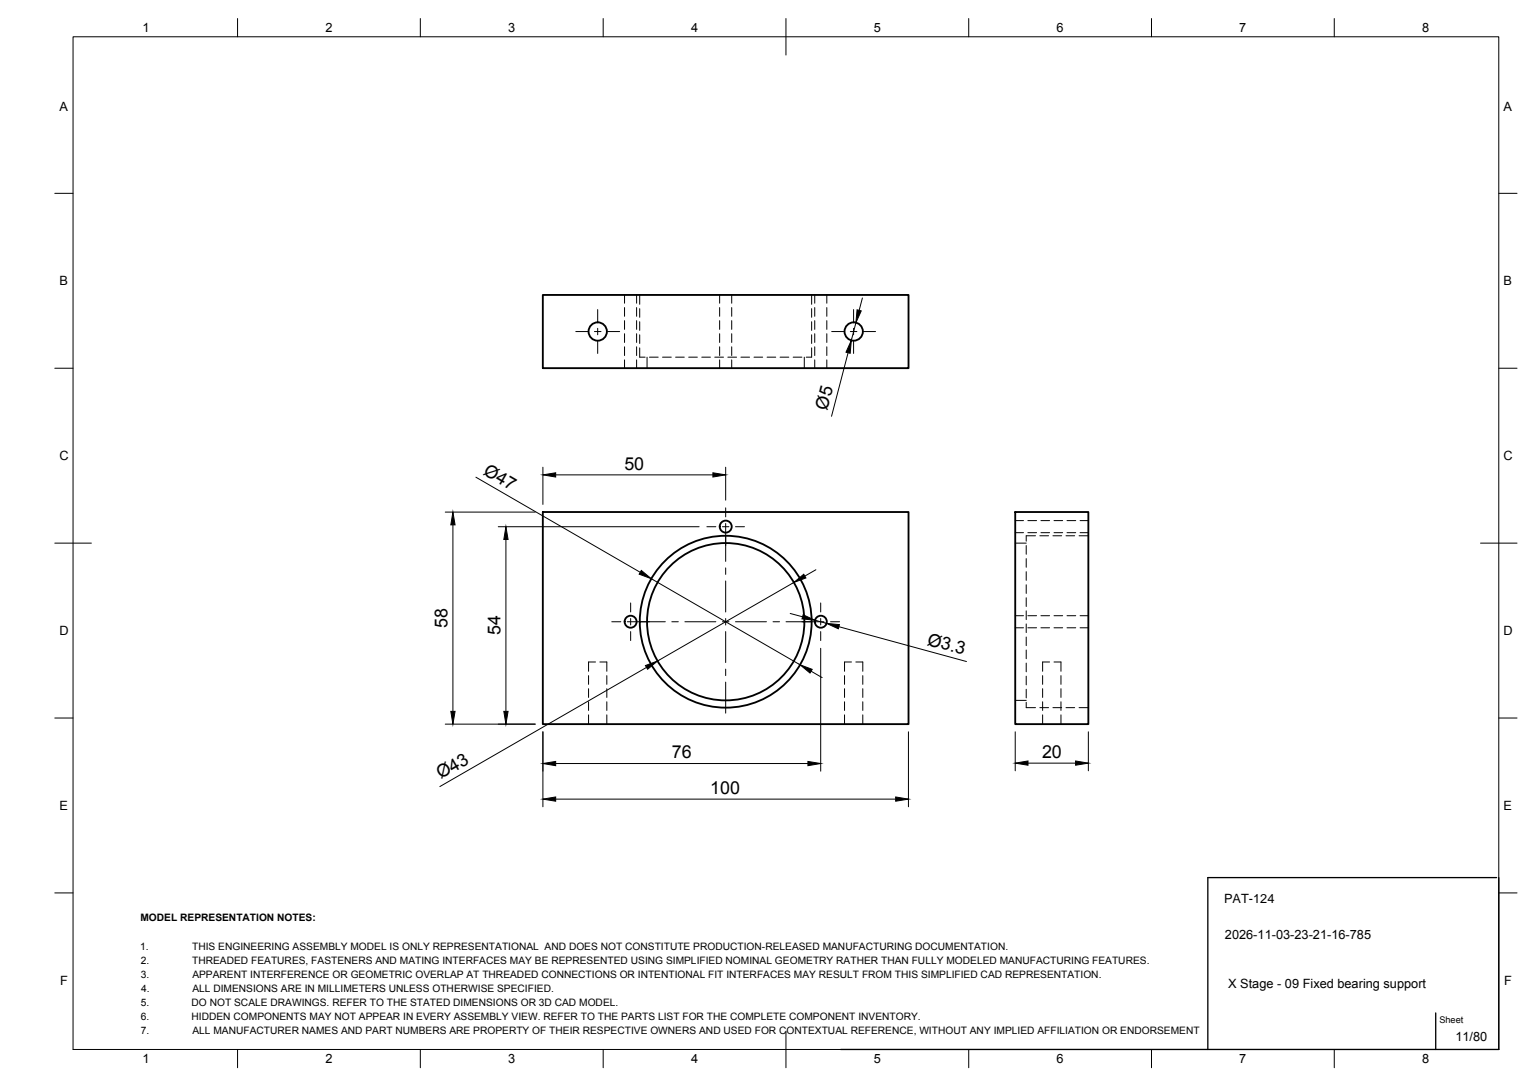
ISO-10303-21;
HEADER;
/* Generated by software containing ST-Developer
 * from STEP Tools, Inc. (www.steptools.com) 
 */

FILE_DESCRIPTION(
/* description */ ('XY cross-slide table'),
/* implementation_level */ '2;1');

FILE_NAME(
/* name */ 'X Stage - 09 Fixed bearing support.step',
/* time_stamp */ '2026-10-28T03:22:46-07:00',
/* author */ (''),
/* organization */ (''),
/* preprocessor_version */ 'ST-DEVELOPER v20.2',
/* originating_system */ 'Autodesk Translation Framework v15.17.0.0',
/* authorisation */ '');

FILE_SCHEMA (('AUTOMOTIVE_DESIGN { 1 0 10303 214 3 1 1 }'));
ENDSEC;

DATA;
#10=MECHANICAL_DESIGN_GEOMETRIC_PRESENTATION_REPRESENTATION('',(#1676),#62984);
#1510=SHAPE_REPRESENTATION_RELATIONSHIP('SRR','None',#63358,#1593);
#1593=ADVANCED_BREP_SHAPE_REPRESENTATION('',(#1789),#62895);
#1676=STYLED_ITEM('',(#63912),#1789);
#1789=MANIFOLD_SOLID_BREP('Body1',#22970);
#1945=FACE_BOUND('',#4323,.T.);
#1946=FACE_BOUND('',#4331,.T.);
#1947=FACE_BOUND('',#4332,.T.);
#1948=FACE_BOUND('',#4333,.T.);
#1949=FACE_BOUND('',#4334,.T.);
#1950=FACE_BOUND('',#4337,.T.);
#1951=FACE_BOUND('',#4338,.T.);
#1952=FACE_BOUND('',#4339,.T.);
#1953=FACE_BOUND('',#4340,.T.);
#1954=FACE_BOUND('',#4343,.T.);
#1955=FACE_BOUND('',#4344,.T.);
#2336=PLANE('',#24173);
#2337=PLANE('',#24180);
#2338=PLANE('',#24184);
#2339=PLANE('',#24185);
#2340=PLANE('',#24186);
#2341=PLANE('',#24187);
#2342=PLANE('',#24188);
#2343=PLANE('',#24189);
#2344=PLANE('',#24190);
#2946=FACE_OUTER_BOUND('',#4318,.T.);
#2947=FACE_OUTER_BOUND('',#4319,.T.);
#2948=FACE_OUTER_BOUND('',#4320,.T.);
#2949=FACE_OUTER_BOUND('',#4321,.T.);
#2950=FACE_OUTER_BOUND('',#4322,.T.);
#2951=FACE_OUTER_BOUND('',#4324,.T.);
#2952=FACE_OUTER_BOUND('',#4325,.T.);
#2953=FACE_OUTER_BOUND('',#4326,.T.);
#2954=FACE_OUTER_BOUND('',#4327,.T.);
#2955=FACE_OUTER_BOUND('',#4328,.T.);
#2956=FACE_OUTER_BOUND('',#4329,.T.);
#2957=FACE_OUTER_BOUND('',#4330,.T.);
#2958=FACE_OUTER_BOUND('',#4335,.T.);
#2959=FACE_OUTER_BOUND('',#4336,.T.);
#2960=FACE_OUTER_BOUND('',#4341,.T.);
#2961=FACE_OUTER_BOUND('',#4342,.T.);
#4318=EDGE_LOOP('',(#15254,#15255,#15256,#15257));
#4319=EDGE_LOOP('',(#15258,#15259,#15260,#15261));
#4320=EDGE_LOOP('',(#15262,#15263,#15264,#15265));
#4321=EDGE_LOOP('',(#15266,#15267,#15268,#15269));
#4322=EDGE_LOOP('',(#15270));
#4323=EDGE_LOOP('',(#15271));
#4324=EDGE_LOOP('',(#15272,#15273,#15274,#15275));
#4325=EDGE_LOOP('',(#15276,#15277,#15278,#15279));
#4326=EDGE_LOOP('',(#15280));
#4327=EDGE_LOOP('',(#15281,#15282,#15283,#15284));
#4328=EDGE_LOOP('',(#15285));
#4329=EDGE_LOOP('',(#15286,#15287,#15288,#15289));
#4330=EDGE_LOOP('',(#15290,#15291,#15292,#15293));
#4331=EDGE_LOOP('',(#15294));
#4332=EDGE_LOOP('',(#15295));
#4333=EDGE_LOOP('',(#15296));
#4334=EDGE_LOOP('',(#15297));
#4335=EDGE_LOOP('',(#15298,#15299,#15300,#15301));
#4336=EDGE_LOOP('',(#15302,#15303,#15304,#15305));
#4337=EDGE_LOOP('',(#15306));
#4338=EDGE_LOOP('',(#15307));
#4339=EDGE_LOOP('',(#15308));
#4340=EDGE_LOOP('',(#15309));
#4341=EDGE_LOOP('',(#15310,#15311,#15312,#15313));
#4342=EDGE_LOOP('',(#15314,#15315,#15316,#15317));
#4343=EDGE_LOOP('',(#15318));
#4344=EDGE_LOOP('',(#15319));
#6007=LINE('',#33250,#7494);
#6008=LINE('',#33256,#7495);
#6009=LINE('',#33262,#7496);
#6010=LINE('',#33268,#7497);
#6011=LINE('',#33276,#7498);
#6012=LINE('',#33281,#7499);
#6013=LINE('',#33288,#7500);
#6014=LINE('',#33294,#7501);
#6015=LINE('',#33296,#7502);
#6016=LINE('',#33298,#7503);
#6017=LINE('',#33299,#7504);
#6018=LINE('',#33302,#7505);
#6019=LINE('',#33304,#7506);
#6020=LINE('',#33305,#7507);
#6021=LINE('',#33308,#7508);
#6022=LINE('',#33310,#7509);
#6023=LINE('',#33311,#7510);
#6024=LINE('',#33313,#7511);
#6025=LINE('',#33314,#7512);
#7494=VECTOR('',#26888,0.165);
#7495=VECTOR('',#26895,0.165);
#7496=VECTOR('',#26902,0.165);
#7497=VECTOR('',#26909,2.35);
#7498=VECTOR('',#26920,2.15);
#7499=VECTOR('',#26925,0.25);
#7500=VECTOR('',#26934,0.25);
#7501=VECTOR('',#26941,1.);
#7502=VECTOR('',#26942,1.);
#7503=VECTOR('',#26943,1.);
#7504=VECTOR('',#26944,1.);
#7505=VECTOR('',#26947,1.);
#7506=VECTOR('',#26948,1.);
#7507=VECTOR('',#26949,1.);
#7508=VECTOR('',#26952,1.);
#7509=VECTOR('',#26953,1.);
#7510=VECTOR('',#26954,1.);
#7511=VECTOR('',#26957,1.);
#7512=VECTOR('',#26958,1.);
#8954=CIRCLE('',#24162,0.165);
#8955=CIRCLE('',#24163,0.165);
#8956=CIRCLE('',#24165,0.165);
#8957=CIRCLE('',#24166,0.165);
#8958=CIRCLE('',#24168,0.165);
#8959=CIRCLE('',#24169,0.165);
#8960=CIRCLE('',#24171,2.35);
#8961=CIRCLE('',#24172,2.35);
#8962=CIRCLE('',#24174,2.15);
#8963=CIRCLE('',#24176,2.15);
#8964=CIRCLE('',#24178,0.25);
#8965=CIRCLE('',#24179,0.25);
#8966=CIRCLE('',#24182,0.25);
#8967=CIRCLE('',#24183,0.25);
#9887=VERTEX_POINT('',#33247);
#9888=VERTEX_POINT('',#33249);
#9889=VERTEX_POINT('',#33253);
#9890=VERTEX_POINT('',#33255);
#9891=VERTEX_POINT('',#33259);
#9892=VERTEX_POINT('',#33261);
#9893=VERTEX_POINT('',#33265);
#9894=VERTEX_POINT('',#33267);
#9895=VERTEX_POINT('',#33271);
#9896=VERTEX_POINT('',#33274);
#9897=VERTEX_POINT('',#33278);
#9898=VERTEX_POINT('',#33280);
#9899=VERTEX_POINT('',#33285);
#9900=VERTEX_POINT('',#33287);
#9901=VERTEX_POINT('',#33292);
#9902=VERTEX_POINT('',#33293);
#9903=VERTEX_POINT('',#33295);
#9904=VERTEX_POINT('',#33297);
#9905=VERTEX_POINT('',#33301);
#9906=VERTEX_POINT('',#33303);
#9907=VERTEX_POINT('',#33307);
#9908=VERTEX_POINT('',#33309);
#12011=EDGE_CURVE('',#9887,#9887,#8954,.T.);
#12012=EDGE_CURVE('',#9887,#9888,#6007,.T.);
#12013=EDGE_CURVE('',#9888,#9888,#8955,.T.);
#12014=EDGE_CURVE('',#9889,#9889,#8956,.T.);
#12015=EDGE_CURVE('',#9889,#9890,#6008,.T.);
#12016=EDGE_CURVE('',#9890,#9890,#8957,.T.);
#12017=EDGE_CURVE('',#9891,#9891,#8958,.T.);
#12018=EDGE_CURVE('',#9891,#9892,#6009,.T.);
#12019=EDGE_CURVE('',#9892,#9892,#8959,.T.);
#12020=EDGE_CURVE('',#9893,#9893,#8960,.T.);
#12021=EDGE_CURVE('',#9893,#9894,#6010,.T.);
#12022=EDGE_CURVE('',#9894,#9894,#8961,.T.);
#12023=EDGE_CURVE('',#9895,#9895,#8962,.T.);
#12024=EDGE_CURVE('',#9896,#9896,#8963,.T.);
#12025=EDGE_CURVE('',#9896,#9895,#6011,.T.);
#12026=EDGE_CURVE('',#9897,#9897,#8964,.T.);
#12027=EDGE_CURVE('',#9897,#9898,#6012,.T.);
#12028=EDGE_CURVE('',#9898,#9898,#8965,.T.);
#12029=EDGE_CURVE('',#9899,#9899,#8966,.T.);
#12030=EDGE_CURVE('',#9899,#9900,#6013,.T.);
#12031=EDGE_CURVE('',#9900,#9900,#8967,.T.);
#12032=EDGE_CURVE('',#9901,#9902,#6014,.T.);
#12033=EDGE_CURVE('',#9902,#9903,#6015,.T.);
#12034=EDGE_CURVE('',#9904,#9903,#6016,.T.);
#12035=EDGE_CURVE('',#9901,#9904,#6017,.T.);
#12036=EDGE_CURVE('',#9905,#9901,#6018,.T.);
#12037=EDGE_CURVE('',#9906,#9904,#6019,.T.);
#12038=EDGE_CURVE('',#9905,#9906,#6020,.T.);
#12039=EDGE_CURVE('',#9907,#9905,#6021,.T.);
#12040=EDGE_CURVE('',#9908,#9906,#6022,.T.);
#12041=EDGE_CURVE('',#9907,#9908,#6023,.T.);
#12042=EDGE_CURVE('',#9902,#9907,#6024,.T.);
#12043=EDGE_CURVE('',#9903,#9908,#6025,.T.);
#15254=ORIENTED_EDGE('',*,*,#12011,.F.);
#15255=ORIENTED_EDGE('',*,*,#12012,.T.);
#15256=ORIENTED_EDGE('',*,*,#12013,.F.);
#15257=ORIENTED_EDGE('',*,*,#12012,.F.);
#15258=ORIENTED_EDGE('',*,*,#12014,.F.);
#15259=ORIENTED_EDGE('',*,*,#12015,.T.);
#15260=ORIENTED_EDGE('',*,*,#12016,.F.);
#15261=ORIENTED_EDGE('',*,*,#12015,.F.);
#15262=ORIENTED_EDGE('',*,*,#12017,.F.);
#15263=ORIENTED_EDGE('',*,*,#12018,.T.);
#15264=ORIENTED_EDGE('',*,*,#12019,.F.);
#15265=ORIENTED_EDGE('',*,*,#12018,.F.);
#15266=ORIENTED_EDGE('',*,*,#12020,.F.);
#15267=ORIENTED_EDGE('',*,*,#12021,.T.);
#15268=ORIENTED_EDGE('',*,*,#12022,.F.);
#15269=ORIENTED_EDGE('',*,*,#12021,.F.);
#15270=ORIENTED_EDGE('',*,*,#12020,.T.);
#15271=ORIENTED_EDGE('',*,*,#12023,.F.);
#15272=ORIENTED_EDGE('',*,*,#12024,.F.);
#15273=ORIENTED_EDGE('',*,*,#12025,.T.);
#15274=ORIENTED_EDGE('',*,*,#12023,.T.);
#15275=ORIENTED_EDGE('',*,*,#12025,.F.);
#15276=ORIENTED_EDGE('',*,*,#12026,.F.);
#15277=ORIENTED_EDGE('',*,*,#12027,.T.);
#15278=ORIENTED_EDGE('',*,*,#12028,.T.);
#15279=ORIENTED_EDGE('',*,*,#12027,.F.);
#15280=ORIENTED_EDGE('',*,*,#12028,.F.);
#15281=ORIENTED_EDGE('',*,*,#12029,.F.);
#15282=ORIENTED_EDGE('',*,*,#12030,.T.);
#15283=ORIENTED_EDGE('',*,*,#12031,.T.);
#15284=ORIENTED_EDGE('',*,*,#12030,.F.);
#15285=ORIENTED_EDGE('',*,*,#12031,.F.);
#15286=ORIENTED_EDGE('',*,*,#12032,.T.);
#15287=ORIENTED_EDGE('',*,*,#12033,.T.);
#15288=ORIENTED_EDGE('',*,*,#12034,.F.);
#15289=ORIENTED_EDGE('',*,*,#12035,.F.);
#15290=ORIENTED_EDGE('',*,*,#12036,.T.);
#15291=ORIENTED_EDGE('',*,*,#12035,.T.);
#15292=ORIENTED_EDGE('',*,*,#12037,.F.);
#15293=ORIENTED_EDGE('',*,*,#12038,.F.);
#15294=ORIENTED_EDGE('',*,*,#12013,.T.);
#15295=ORIENTED_EDGE('',*,*,#12016,.T.);
#15296=ORIENTED_EDGE('',*,*,#12019,.T.);
#15297=ORIENTED_EDGE('',*,*,#12022,.T.);
#15298=ORIENTED_EDGE('',*,*,#12039,.T.);
#15299=ORIENTED_EDGE('',*,*,#12038,.T.);
#15300=ORIENTED_EDGE('',*,*,#12040,.F.);
#15301=ORIENTED_EDGE('',*,*,#12041,.F.);
#15302=ORIENTED_EDGE('',*,*,#12042,.T.);
#15303=ORIENTED_EDGE('',*,*,#12041,.T.);
#15304=ORIENTED_EDGE('',*,*,#12043,.F.);
#15305=ORIENTED_EDGE('',*,*,#12033,.F.);
#15306=ORIENTED_EDGE('',*,*,#12011,.T.);
#15307=ORIENTED_EDGE('',*,*,#12014,.T.);
#15308=ORIENTED_EDGE('',*,*,#12017,.T.);
#15309=ORIENTED_EDGE('',*,*,#12024,.T.);
#15310=ORIENTED_EDGE('',*,*,#12043,.T.);
#15311=ORIENTED_EDGE('',*,*,#12040,.T.);
#15312=ORIENTED_EDGE('',*,*,#12037,.T.);
#15313=ORIENTED_EDGE('',*,*,#12034,.T.);
#15314=ORIENTED_EDGE('',*,*,#12042,.F.);
#15315=ORIENTED_EDGE('',*,*,#12032,.F.);
#15316=ORIENTED_EDGE('',*,*,#12036,.F.);
#15317=ORIENTED_EDGE('',*,*,#12039,.F.);
#15318=ORIENTED_EDGE('',*,*,#12026,.T.);
#15319=ORIENTED_EDGE('',*,*,#12029,.T.);
#21077=CYLINDRICAL_SURFACE('',#24161,0.165);
#21078=CYLINDRICAL_SURFACE('',#24164,0.165);
#21079=CYLINDRICAL_SURFACE('',#24167,0.165);
#21080=CYLINDRICAL_SURFACE('',#24170,2.35);
#21081=CYLINDRICAL_SURFACE('',#24175,2.15);
#21082=CYLINDRICAL_SURFACE('',#24177,0.25);
#21083=CYLINDRICAL_SURFACE('',#24181,0.25);
#21727=ADVANCED_FACE('',(#2946),#21077,.F.);
#21728=ADVANCED_FACE('',(#2947),#21078,.F.);
#21729=ADVANCED_FACE('',(#2948),#21079,.F.);
#21730=ADVANCED_FACE('',(#2949),#21080,.F.);
#21731=ADVANCED_FACE('',(#2950,#1945),#2336,.T.);
#21732=ADVANCED_FACE('',(#2951),#21081,.F.);
#21733=ADVANCED_FACE('',(#2952),#21082,.F.);
#21734=ADVANCED_FACE('',(#2953),#2337,.F.);
#21735=ADVANCED_FACE('',(#2954),#21083,.F.);
#21736=ADVANCED_FACE('',(#2955),#2338,.F.);
#21737=ADVANCED_FACE('',(#2956),#2339,.T.);
#21738=ADVANCED_FACE('',(#2957,#1946,#1947,#1948,#1949),#2340,.T.);
#21739=ADVANCED_FACE('',(#2958),#2341,.T.);
#21740=ADVANCED_FACE('',(#2959,#1950,#1951,#1952,#1953),#2342,.T.);
#21741=ADVANCED_FACE('',(#2960),#2343,.T.);
#21742=ADVANCED_FACE('',(#2961,#1954,#1955),#2344,.F.);
#22970=CLOSED_SHELL('',(#21727,#21728,#21729,#21730,#21731,#21732,#21733,
#21734,#21735,#21736,#21737,#21738,#21739,#21740,#21741,#21742));
#24160=AXIS2_PLACEMENT_3D('',#33245,#26882,#26883);
#24161=AXIS2_PLACEMENT_3D('',#33246,#26884,#26885);
#24162=AXIS2_PLACEMENT_3D('',#33248,#26886,#26887);
#24163=AXIS2_PLACEMENT_3D('',#33251,#26889,#26890);
#24164=AXIS2_PLACEMENT_3D('',#33252,#26891,#26892);
#24165=AXIS2_PLACEMENT_3D('',#33254,#26893,#26894);
#24166=AXIS2_PLACEMENT_3D('',#33257,#26896,#26897);
#24167=AXIS2_PLACEMENT_3D('',#33258,#26898,#26899);
#24168=AXIS2_PLACEMENT_3D('',#33260,#26900,#26901);
#24169=AXIS2_PLACEMENT_3D('',#33263,#26903,#26904);
#24170=AXIS2_PLACEMENT_3D('',#33264,#26905,#26906);
#24171=AXIS2_PLACEMENT_3D('',#33266,#26907,#26908);
#24172=AXIS2_PLACEMENT_3D('',#33269,#26910,#26911);
#24173=AXIS2_PLACEMENT_3D('',#33270,#26912,#26913);
#24174=AXIS2_PLACEMENT_3D('',#33272,#26914,#26915);
#24175=AXIS2_PLACEMENT_3D('',#33273,#26916,#26917);
#24176=AXIS2_PLACEMENT_3D('',#33275,#26918,#26919);
#24177=AXIS2_PLACEMENT_3D('',#33277,#26921,#26922);
#24178=AXIS2_PLACEMENT_3D('',#33279,#26923,#26924);
#24179=AXIS2_PLACEMENT_3D('',#33282,#26926,#26927);
#24180=AXIS2_PLACEMENT_3D('',#33283,#26928,#26929);
#24181=AXIS2_PLACEMENT_3D('',#33284,#26930,#26931);
#24182=AXIS2_PLACEMENT_3D('',#33286,#26932,#26933);
#24183=AXIS2_PLACEMENT_3D('',#33289,#26935,#26936);
#24184=AXIS2_PLACEMENT_3D('',#33290,#26937,#26938);
#24185=AXIS2_PLACEMENT_3D('',#33291,#26939,#26940);
#24186=AXIS2_PLACEMENT_3D('',#33300,#26945,#26946);
#24187=AXIS2_PLACEMENT_3D('',#33306,#26950,#26951);
#24188=AXIS2_PLACEMENT_3D('',#33312,#26955,#26956);
#24189=AXIS2_PLACEMENT_3D('',#33315,#26959,#26960);
#24190=AXIS2_PLACEMENT_3D('',#33316,#26961,#26962);
#26882=DIRECTION('axis',(0.,0.,1.));
#26883=DIRECTION('refdir',(1.,0.,0.));
#26884=DIRECTION('center_axis',(1.,0.,0.));
#26885=DIRECTION('ref_axis',(0.,0.,-1.));
#26886=DIRECTION('center_axis',(1.,0.,0.));
#26887=DIRECTION('ref_axis',(0.,0.,-1.));
#26888=DIRECTION('',(1.,0.,0.));
#26889=DIRECTION('center_axis',(-1.,0.,0.));
#26890=DIRECTION('ref_axis',(0.,0.,-1.));
#26891=DIRECTION('center_axis',(1.,0.,0.));
#26892=DIRECTION('ref_axis',(0.,0.,-1.));
#26893=DIRECTION('center_axis',(1.,0.,0.));
#26894=DIRECTION('ref_axis',(0.,0.,-1.));
#26895=DIRECTION('',(1.,0.,0.));
#26896=DIRECTION('center_axis',(-1.,0.,0.));
#26897=DIRECTION('ref_axis',(0.,0.,-1.));
#26898=DIRECTION('center_axis',(1.,0.,0.));
#26899=DIRECTION('ref_axis',(0.,0.,-1.));
#26900=DIRECTION('center_axis',(1.,0.,0.));
#26901=DIRECTION('ref_axis',(0.,0.,-1.));
#26902=DIRECTION('',(1.,0.,0.));
#26903=DIRECTION('center_axis',(-1.,0.,0.));
#26904=DIRECTION('ref_axis',(0.,0.,-1.));
#26905=DIRECTION('center_axis',(1.,0.,0.));
#26906=DIRECTION('ref_axis',(0.,0.,-1.));
#26907=DIRECTION('center_axis',(1.,0.,0.));
#26908=DIRECTION('ref_axis',(0.,0.,-1.));
#26909=DIRECTION('',(1.,0.,0.));
#26910=DIRECTION('center_axis',(-1.,0.,0.));
#26911=DIRECTION('ref_axis',(0.,0.,-1.));
#26912=DIRECTION('center_axis',(1.,0.,0.));
#26913=DIRECTION('ref_axis',(0.,0.,-1.));
#26914=DIRECTION('center_axis',(1.,0.,0.));
#26915=DIRECTION('ref_axis',(0.,0.,-1.));
#26916=DIRECTION('center_axis',(1.,0.,0.));
#26917=DIRECTION('ref_axis',(0.,0.,-1.));
#26918=DIRECTION('center_axis',(1.,0.,0.));
#26919=DIRECTION('ref_axis',(0.,0.,-1.));
#26920=DIRECTION('',(1.,0.,0.));
#26921=DIRECTION('center_axis',(0.,0.,1.));
#26922=DIRECTION('ref_axis',(1.,0.,0.));
#26923=DIRECTION('center_axis',(0.,0.,1.));
#26924=DIRECTION('ref_axis',(1.,0.,0.));
#26925=DIRECTION('',(0.,0.,1.));
#26926=DIRECTION('center_axis',(0.,0.,1.));
#26927=DIRECTION('ref_axis',(1.,0.,0.));
#26928=DIRECTION('center_axis',(0.,0.,1.));
#26929=DIRECTION('ref_axis',(1.,0.,0.));
#26930=DIRECTION('center_axis',(0.,0.,1.));
#26931=DIRECTION('ref_axis',(1.,0.,0.));
#26932=DIRECTION('center_axis',(0.,0.,1.));
#26933=DIRECTION('ref_axis',(1.,0.,0.));
#26934=DIRECTION('',(0.,0.,1.));
#26935=DIRECTION('center_axis',(0.,0.,1.));
#26936=DIRECTION('ref_axis',(1.,0.,0.));
#26937=DIRECTION('center_axis',(0.,0.,1.));
#26938=DIRECTION('ref_axis',(1.,0.,0.));
#26939=DIRECTION('center_axis',(0.,1.,0.));
#26940=DIRECTION('ref_axis',(-1.,0.,0.));
#26941=DIRECTION('',(-1.,0.,0.));
#26942=DIRECTION('',(0.,0.,1.));
#26943=DIRECTION('',(-1.,0.,0.));
#26944=DIRECTION('',(0.,0.,1.));
#26945=DIRECTION('center_axis',(1.,0.,0.));
#26946=DIRECTION('ref_axis',(0.,1.,0.));
#26947=DIRECTION('',(0.,1.,0.));
#26948=DIRECTION('',(0.,1.,0.));
#26949=DIRECTION('',(0.,0.,1.));
#26950=DIRECTION('center_axis',(0.,-1.,0.));
#26951=DIRECTION('ref_axis',(1.,0.,0.));
#26952=DIRECTION('',(1.,0.,0.));
#26953=DIRECTION('',(1.,0.,0.));
#26954=DIRECTION('',(0.,0.,1.));
#26955=DIRECTION('center_axis',(-1.,0.,0.));
#26956=DIRECTION('ref_axis',(0.,-1.,0.));
#26957=DIRECTION('',(0.,-1.,0.));
#26958=DIRECTION('',(0.,-1.,0.));
#26959=DIRECTION('center_axis',(0.,0.,1.));
#26960=DIRECTION('ref_axis',(1.,0.,0.));
#26961=DIRECTION('center_axis',(0.,0.,1.));
#26962=DIRECTION('ref_axis',(1.,0.,0.));
#33245=CARTESIAN_POINT('',(0.,0.,0.));
#33246=CARTESIAN_POINT('Origin',(22.9,-2.6,4.));
#33247=CARTESIAN_POINT('',(23.,-2.6,4.165));
#33248=CARTESIAN_POINT('Origin',(23.,-2.6,4.));
#33249=CARTESIAN_POINT('',(25.,-2.6,4.165));
#33250=CARTESIAN_POINT('',(22.9,-2.6,4.165));
#33251=CARTESIAN_POINT('Origin',(25.,-2.6,4.));
#33252=CARTESIAN_POINT('Origin',(22.9,2.6,4.));
#33253=CARTESIAN_POINT('',(23.,2.6,4.165));
#33254=CARTESIAN_POINT('Origin',(23.,2.6,4.));
#33255=CARTESIAN_POINT('',(25.,2.6,4.165));
#33256=CARTESIAN_POINT('',(22.9,2.6,4.165));
#33257=CARTESIAN_POINT('Origin',(25.,2.6,4.));
#33258=CARTESIAN_POINT('Origin',(22.9,0.,6.6));
#33259=CARTESIAN_POINT('',(23.,-2.02066721859313E-17,6.765));
#33260=CARTESIAN_POINT('Origin',(23.,0.,6.6));
#33261=CARTESIAN_POINT('',(25.,2.02066721859313E-17,6.765));
#33262=CARTESIAN_POINT('',(22.9,-2.02066721859313E-17,6.765));
#33263=CARTESIAN_POINT('Origin',(25.,0.,6.6));
#33264=CARTESIAN_POINT('Origin',(23.3,0.,4.));
#33265=CARTESIAN_POINT('',(23.3,-2.87791997799628E-16,6.35));
#33266=CARTESIAN_POINT('Origin',(23.3,0.,4.));
#33267=CARTESIAN_POINT('',(25.,2.87791997799628E-16,6.35));
#33268=CARTESIAN_POINT('',(23.3,-2.87791997799628E-16,6.35));
#33269=CARTESIAN_POINT('Origin',(25.,0.,4.));
#33270=CARTESIAN_POINT('Origin',(23.3,0.,4.));
#33271=CARTESIAN_POINT('',(23.3,-2.63299061816681E-16,6.15));
#33272=CARTESIAN_POINT('Origin',(23.3,0.,4.));
#33273=CARTESIAN_POINT('Origin',(22.9,0.,4.));
#33274=CARTESIAN_POINT('',(23.,-2.63299061816681E-16,6.15));
#33275=CARTESIAN_POINT('Origin',(23.,0.,4.));
#33276=CARTESIAN_POINT('',(22.9,-2.63299061816681E-16,6.15));
#33277=CARTESIAN_POINT('Origin',(24.,-3.5,1.1));
#33278=CARTESIAN_POINT('',(23.75,-3.5,1.2));
#33279=CARTESIAN_POINT('Origin',(24.,-3.5,1.2));
#33280=CARTESIAN_POINT('',(23.75,-3.5,2.9));
#33281=CARTESIAN_POINT('',(23.75,-3.5,1.1));
#33282=CARTESIAN_POINT('Origin',(24.,-3.5,2.9));
#33283=CARTESIAN_POINT('Origin',(24.,-3.5,2.9));
#33284=CARTESIAN_POINT('Origin',(24.,3.5,1.1));
#33285=CARTESIAN_POINT('',(23.75,3.5,1.2));
#33286=CARTESIAN_POINT('Origin',(24.,3.5,1.2));
#33287=CARTESIAN_POINT('',(23.75,3.5,2.9));
#33288=CARTESIAN_POINT('',(23.75,3.5,1.1));
#33289=CARTESIAN_POINT('Origin',(24.,3.5,2.9));
#33290=CARTESIAN_POINT('Origin',(24.,3.5,2.9));
#33291=CARTESIAN_POINT('Origin',(25.,5.,1.2));
#33292=CARTESIAN_POINT('',(25.,5.,1.2));
#33293=CARTESIAN_POINT('',(23.,5.,1.2));
#33294=CARTESIAN_POINT('',(25.,5.,1.2));
#33295=CARTESIAN_POINT('',(23.,5.,7.));
#33296=CARTESIAN_POINT('',(23.,5.,1.2));
#33297=CARTESIAN_POINT('',(25.,5.,7.));
#33298=CARTESIAN_POINT('',(25.,5.,7.));
#33299=CARTESIAN_POINT('',(25.,5.,1.2));
#33300=CARTESIAN_POINT('Origin',(25.,-5.,1.2));
#33301=CARTESIAN_POINT('',(25.,-5.,1.2));
#33302=CARTESIAN_POINT('',(25.,-5.,1.2));
#33303=CARTESIAN_POINT('',(25.,-5.,7.));
#33304=CARTESIAN_POINT('',(25.,-5.,7.));
#33305=CARTESIAN_POINT('',(25.,-5.,1.2));
#33306=CARTESIAN_POINT('Origin',(23.,-5.,1.2));
#33307=CARTESIAN_POINT('',(23.,-5.,1.2));
#33308=CARTESIAN_POINT('',(23.,-5.,1.2));
#33309=CARTESIAN_POINT('',(23.,-5.,7.));
#33310=CARTESIAN_POINT('',(23.,-5.,7.));
#33311=CARTESIAN_POINT('',(23.,-5.,1.2));
#33312=CARTESIAN_POINT('Origin',(23.,5.,1.2));
#33313=CARTESIAN_POINT('',(23.,5.,1.2));
#33314=CARTESIAN_POINT('',(23.,5.,7.));
#33315=CARTESIAN_POINT('Origin',(24.,0.,7.));
#33316=CARTESIAN_POINT('Origin',(24.,0.,1.2));
#62796=UNCERTAINTY_MEASURE_WITH_UNIT(LENGTH_MEASURE(0.001),#62985,
'DISTANCE_ACCURACY_VALUE',
'Maximum model space distance between geometric entities at asserted c
onnectivities');
#62885=UNCERTAINTY_MEASURE_WITH_UNIT(LENGTH_MEASURE(0.001),#62985,
'DISTANCE_ACCURACY_VALUE',
'Maximum model space distance between geometric entities at asserted c
onnectivities');
#62895=(
GEOMETRIC_REPRESENTATION_CONTEXT(3)
GLOBAL_UNCERTAINTY_ASSIGNED_CONTEXT((#62796))
GLOBAL_UNIT_ASSIGNED_CONTEXT((#62985,#62987,#62988))
REPRESENTATION_CONTEXT('','3D')
);
#62984=(
GEOMETRIC_REPRESENTATION_CONTEXT(3)
GLOBAL_UNCERTAINTY_ASSIGNED_CONTEXT((#62885))
GLOBAL_UNIT_ASSIGNED_CONTEXT((#62985,#62987,#62988))
REPRESENTATION_CONTEXT('','3D')
);
#62985=(
LENGTH_UNIT()
NAMED_UNIT(*)
SI_UNIT(.CENTI.,.METRE.)
);
#62987=(
NAMED_UNIT(*)
PLANE_ANGLE_UNIT()
SI_UNIT($,.RADIAN.)
);
#62988=(
NAMED_UNIT(*)
SI_UNIT($,.STERADIAN.)
SOLID_ANGLE_UNIT()
);
#62998=SHAPE_DEFINITION_REPRESENTATION(#63096,#63358);
#63096=PRODUCT_DEFINITION_SHAPE('',$,#63457);
#63358=SHAPE_REPRESENTATION('',(#24160),#62895);
#63447=PRODUCT_DEFINITION_CONTEXT('part definition',#63743,'design');
#63457=PRODUCT_DEFINITION('X Stage - 09 Fixed bearing support',
'X Stage - 09 Fixed bearing support',#63555,#63447);
#63555=PRODUCT_DEFINITION_FORMATION('',$,#63754);
#63743=APPLICATION_CONTEXT(
'Core Data for Automotive Mechanical Design Process');
#63744=PRODUCT_CONTEXT('part definition',#63743,'mechanical');
#63754=PRODUCT('X Stage - 09 Fixed bearing support',
'X Stage - 09 Fixed bearing support',
'X Stage - 09 Fixed bearing support',(#63744));
#63906=COLOUR_RGB('Grey',0.48,0.52,0.57);
#63907=FILL_AREA_STYLE_COLOUR('',#63906);
#63908=FILL_AREA_STYLE('',(#63907));
#63909=SURFACE_STYLE_FILL_AREA(#63908);
#63910=SURFACE_SIDE_STYLE('',(#63909));
#63911=SURFACE_STYLE_USAGE(.BOTH.,#63910);
#63912=PRESENTATION_STYLE_ASSIGNMENT((#63911));
ENDSEC;
END-ISO-10303-21;
